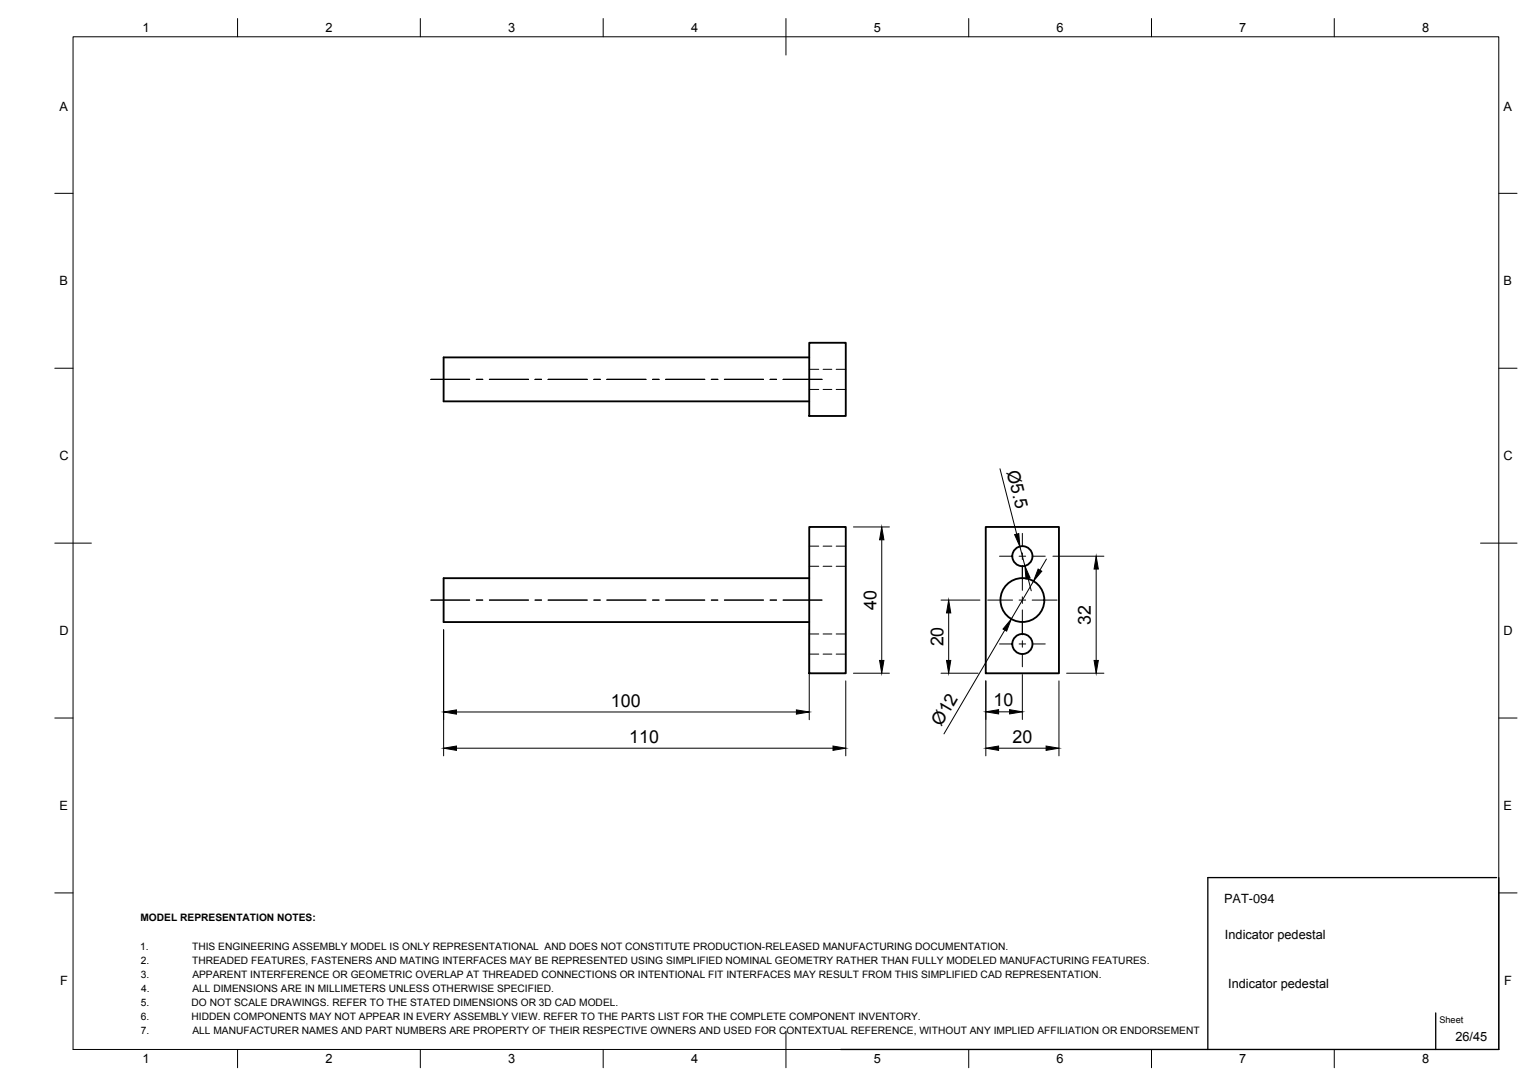
ISO-10303-21;
HEADER;
/* Generated by software containing ST-Developer
 * from STEP Tools, Inc. (www.steptools.com) 
 */

FILE_DESCRIPTION(
/* description */ ('Shaft runout checking stand'),
/* implementation_level */ '2;1');

FILE_NAME(
/* name */ 'Indicator pedestal.step',
/* time_stamp */ '2026-11-02T21:12:33-08:00',
/* author */ (''),
/* organization */ (''),
/* preprocessor_version */ 'ST-DEVELOPER v20.2',
/* originating_system */ 'Autodesk Translation Framework v15.17.0.0',
/* authorisation */ '');

FILE_SCHEMA (('AUTOMOTIVE_DESIGN { 1 0 10303 214 3 1 1 }'));
ENDSEC;

DATA;
#10=MECHANICAL_DESIGN_GEOMETRIC_PRESENTATION_REPRESENTATION('',(#486),#11748);
#400=SHAPE_REPRESENTATION_RELATIONSHIP('SRR','None',#11949,#443);
#443=ADVANCED_BREP_SHAPE_REPRESENTATION('',(#535),#11725);
#486=STYLED_ITEM('',(#12169),#535);
#535=MANIFOLD_SOLID_BREP('Body1',#6231);
#635=FACE_BOUND('',#1708,.T.);
#636=FACE_BOUND('',#1709,.T.);
#637=FACE_BOUND('',#1710,.T.);
#638=FACE_BOUND('',#1712,.T.);
#639=FACE_BOUND('',#1713,.T.);
#802=CIRCLE('',#7112,0.6);
#803=CIRCLE('',#7113,0.6);
#804=CIRCLE('',#7116,0.275);
#805=CIRCLE('',#7117,0.275);
#806=CIRCLE('',#7119,0.275);
#807=CIRCLE('',#7120,0.275);
#998=CYLINDRICAL_SURFACE('',#7111,0.6);
#999=CYLINDRICAL_SURFACE('',#7115,0.275);
#1000=CYLINDRICAL_SURFACE('',#7118,0.275);
#1258=FACE_OUTER_BOUND('',#1699,.T.);
#1259=FACE_OUTER_BOUND('',#1700,.T.);
#1260=FACE_OUTER_BOUND('',#1701,.T.);
#1261=FACE_OUTER_BOUND('',#1702,.T.);
#1262=FACE_OUTER_BOUND('',#1703,.T.);
#1263=FACE_OUTER_BOUND('',#1704,.T.);
#1264=FACE_OUTER_BOUND('',#1705,.T.);
#1265=FACE_OUTER_BOUND('',#1706,.T.);
#1266=FACE_OUTER_BOUND('',#1707,.T.);
#1267=FACE_OUTER_BOUND('',#1711,.T.);
#1699=EDGE_LOOP('',(#5040,#5041,#5042,#5043));
#1700=EDGE_LOOP('',(#5044));
#1701=EDGE_LOOP('',(#5045,#5046,#5047,#5048));
#1702=EDGE_LOOP('',(#5049,#5050,#5051,#5052));
#1703=EDGE_LOOP('',(#5053,#5054,#5055,#5056));
#1704=EDGE_LOOP('',(#5057,#5058,#5059,#5060));
#1705=EDGE_LOOP('',(#5061,#5062,#5063,#5064));
#1706=EDGE_LOOP('',(#5065,#5066,#5067,#5068));
#1707=EDGE_LOOP('',(#5069,#5070,#5071,#5072));
#1708=EDGE_LOOP('',(#5073));
#1709=EDGE_LOOP('',(#5074));
#1710=EDGE_LOOP('',(#5075));
#1711=EDGE_LOOP('',(#5076,#5077,#5078,#5079));
#1712=EDGE_LOOP('',(#5080));
#1713=EDGE_LOOP('',(#5081));
#2230=LINE('',#10516,#2697);
#2231=LINE('',#10523,#2698);
#2232=LINE('',#10529,#2699);
#2233=LINE('',#10534,#2700);
#2234=LINE('',#10536,#2701);
#2235=LINE('',#10538,#2702);
#2236=LINE('',#10539,#2703);
#2237=LINE('',#10542,#2704);
#2238=LINE('',#10544,#2705);
#2239=LINE('',#10545,#2706);
#2240=LINE('',#10548,#2707);
#2241=LINE('',#10550,#2708);
#2242=LINE('',#10551,#2709);
#2243=LINE('',#10553,#2710);
#2244=LINE('',#10554,#2711);
#2697=VECTOR('',#8595,0.6);
#2698=VECTOR('',#8604,0.275);
#2699=VECTOR('',#8611,0.275);
#2700=VECTOR('',#8616,1.);
#2701=VECTOR('',#8617,1.);
#2702=VECTOR('',#8618,1.);
#2703=VECTOR('',#8619,1.);
#2704=VECTOR('',#8622,1.);
#2705=VECTOR('',#8623,1.);
#2706=VECTOR('',#8624,1.);
#2707=VECTOR('',#8627,1.);
#2708=VECTOR('',#8628,1.);
#2709=VECTOR('',#8629,1.);
#2710=VECTOR('',#8632,1.);
#2711=VECTOR('',#8633,1.);
#3134=VERTEX_POINT('',#10513);
#3135=VERTEX_POINT('',#10515);
#3136=VERTEX_POINT('',#10520);
#3137=VERTEX_POINT('',#10522);
#3138=VERTEX_POINT('',#10526);
#3139=VERTEX_POINT('',#10528);
#3140=VERTEX_POINT('',#10532);
#3141=VERTEX_POINT('',#10533);
#3142=VERTEX_POINT('',#10535);
#3143=VERTEX_POINT('',#10537);
#3144=VERTEX_POINT('',#10541);
#3145=VERTEX_POINT('',#10543);
#3146=VERTEX_POINT('',#10547);
#3147=VERTEX_POINT('',#10549);
#3806=EDGE_CURVE('',#3134,#3134,#802,.T.);
#3807=EDGE_CURVE('',#3134,#3135,#2230,.T.);
#3808=EDGE_CURVE('',#3135,#3135,#803,.T.);
#3809=EDGE_CURVE('',#3136,#3136,#804,.T.);
#3810=EDGE_CURVE('',#3136,#3137,#2231,.T.);
#3811=EDGE_CURVE('',#3137,#3137,#805,.T.);
#3812=EDGE_CURVE('',#3138,#3138,#806,.T.);
#3813=EDGE_CURVE('',#3138,#3139,#2232,.T.);
#3814=EDGE_CURVE('',#3139,#3139,#807,.T.);
#3815=EDGE_CURVE('',#3140,#3141,#2233,.T.);
#3816=EDGE_CURVE('',#3141,#3142,#2234,.T.);
#3817=EDGE_CURVE('',#3143,#3142,#2235,.T.);
#3818=EDGE_CURVE('',#3140,#3143,#2236,.T.);
#3819=EDGE_CURVE('',#3144,#3140,#2237,.T.);
#3820=EDGE_CURVE('',#3145,#3143,#2238,.T.);
#3821=EDGE_CURVE('',#3144,#3145,#2239,.T.);
#3822=EDGE_CURVE('',#3146,#3144,#2240,.T.);
#3823=EDGE_CURVE('',#3147,#3145,#2241,.T.);
#3824=EDGE_CURVE('',#3146,#3147,#2242,.T.);
#3825=EDGE_CURVE('',#3141,#3146,#2243,.T.);
#3826=EDGE_CURVE('',#3142,#3147,#2244,.T.);
#5040=ORIENTED_EDGE('',*,*,#3806,.F.);
#5041=ORIENTED_EDGE('',*,*,#3807,.T.);
#5042=ORIENTED_EDGE('',*,*,#3808,.F.);
#5043=ORIENTED_EDGE('',*,*,#3807,.F.);
#5044=ORIENTED_EDGE('',*,*,#3806,.T.);
#5045=ORIENTED_EDGE('',*,*,#3809,.F.);
#5046=ORIENTED_EDGE('',*,*,#3810,.T.);
#5047=ORIENTED_EDGE('',*,*,#3811,.F.);
#5048=ORIENTED_EDGE('',*,*,#3810,.F.);
#5049=ORIENTED_EDGE('',*,*,#3812,.F.);
#5050=ORIENTED_EDGE('',*,*,#3813,.T.);
#5051=ORIENTED_EDGE('',*,*,#3814,.F.);
#5052=ORIENTED_EDGE('',*,*,#3813,.F.);
#5053=ORIENTED_EDGE('',*,*,#3815,.T.);
#5054=ORIENTED_EDGE('',*,*,#3816,.T.);
#5055=ORIENTED_EDGE('',*,*,#3817,.F.);
#5056=ORIENTED_EDGE('',*,*,#3818,.F.);
#5057=ORIENTED_EDGE('',*,*,#3819,.T.);
#5058=ORIENTED_EDGE('',*,*,#3818,.T.);
#5059=ORIENTED_EDGE('',*,*,#3820,.F.);
#5060=ORIENTED_EDGE('',*,*,#3821,.F.);
#5061=ORIENTED_EDGE('',*,*,#3822,.T.);
#5062=ORIENTED_EDGE('',*,*,#3821,.T.);
#5063=ORIENTED_EDGE('',*,*,#3823,.F.);
#5064=ORIENTED_EDGE('',*,*,#3824,.F.);
#5065=ORIENTED_EDGE('',*,*,#3825,.T.);
#5066=ORIENTED_EDGE('',*,*,#3824,.T.);
#5067=ORIENTED_EDGE('',*,*,#3826,.F.);
#5068=ORIENTED_EDGE('',*,*,#3816,.F.);
#5069=ORIENTED_EDGE('',*,*,#3826,.T.);
#5070=ORIENTED_EDGE('',*,*,#3823,.T.);
#5071=ORIENTED_EDGE('',*,*,#3820,.T.);
#5072=ORIENTED_EDGE('',*,*,#3817,.T.);
#5073=ORIENTED_EDGE('',*,*,#3808,.T.);
#5074=ORIENTED_EDGE('',*,*,#3811,.T.);
#5075=ORIENTED_EDGE('',*,*,#3814,.T.);
#5076=ORIENTED_EDGE('',*,*,#3825,.F.);
#5077=ORIENTED_EDGE('',*,*,#3815,.F.);
#5078=ORIENTED_EDGE('',*,*,#3819,.F.);
#5079=ORIENTED_EDGE('',*,*,#3822,.F.);
#5080=ORIENTED_EDGE('',*,*,#3809,.T.);
#5081=ORIENTED_EDGE('',*,*,#3812,.T.);
#5757=PLANE('',#7114);
#5758=PLANE('',#7121);
#5759=PLANE('',#7122);
#5760=PLANE('',#7123);
#5761=PLANE('',#7124);
#5762=PLANE('',#7125);
#5763=PLANE('',#7126);
#6058=ADVANCED_FACE('',(#1258),#998,.T.);
#6059=ADVANCED_FACE('',(#1259),#5757,.T.);
#6060=ADVANCED_FACE('',(#1260),#999,.F.);
#6061=ADVANCED_FACE('',(#1261),#1000,.F.);
#6062=ADVANCED_FACE('',(#1262),#5758,.T.);
#6063=ADVANCED_FACE('',(#1263),#5759,.T.);
#6064=ADVANCED_FACE('',(#1264),#5760,.T.);
#6065=ADVANCED_FACE('',(#1265),#5761,.T.);
#6066=ADVANCED_FACE('',(#1266,#635,#636,#637),#5762,.T.);
#6067=ADVANCED_FACE('',(#1267,#638,#639),#5763,.F.);
#6231=CLOSED_SHELL('',(#6058,#6059,#6060,#6061,#6062,#6063,#6064,#6065,
#6066,#6067));
#7110=AXIS2_PLACEMENT_3D('',#10511,#8589,#8590);
#7111=AXIS2_PLACEMENT_3D('',#10512,#8591,#8592);
#7112=AXIS2_PLACEMENT_3D('',#10514,#8593,#8594);
#7113=AXIS2_PLACEMENT_3D('',#10517,#8596,#8597);
#7114=AXIS2_PLACEMENT_3D('',#10518,#8598,#8599);
#7115=AXIS2_PLACEMENT_3D('',#10519,#8600,#8601);
#7116=AXIS2_PLACEMENT_3D('',#10521,#8602,#8603);
#7117=AXIS2_PLACEMENT_3D('',#10524,#8605,#8606);
#7118=AXIS2_PLACEMENT_3D('',#10525,#8607,#8608);
#7119=AXIS2_PLACEMENT_3D('',#10527,#8609,#8610);
#7120=AXIS2_PLACEMENT_3D('',#10530,#8612,#8613);
#7121=AXIS2_PLACEMENT_3D('',#10531,#8614,#8615);
#7122=AXIS2_PLACEMENT_3D('',#10540,#8620,#8621);
#7123=AXIS2_PLACEMENT_3D('',#10546,#8625,#8626);
#7124=AXIS2_PLACEMENT_3D('',#10552,#8630,#8631);
#7125=AXIS2_PLACEMENT_3D('',#10555,#8634,#8635);
#7126=AXIS2_PLACEMENT_3D('',#10556,#8636,#8637);
#8589=DIRECTION('axis',(0.,0.,1.));
#8590=DIRECTION('refdir',(1.,0.,0.));
#8591=DIRECTION('center_axis',(0.,0.,1.));
#8592=DIRECTION('ref_axis',(1.,0.,0.));
#8593=DIRECTION('center_axis',(0.,0.,1.));
#8594=DIRECTION('ref_axis',(1.,0.,0.));
#8595=DIRECTION('',(0.,0.,-1.));
#8596=DIRECTION('center_axis',(0.,0.,-1.));
#8597=DIRECTION('ref_axis',(1.,0.,0.));
#8598=DIRECTION('center_axis',(0.,0.,1.));
#8599=DIRECTION('ref_axis',(1.,0.,0.));
#8600=DIRECTION('center_axis',(0.,0.,1.));
#8601=DIRECTION('ref_axis',(1.,0.,0.));
#8602=DIRECTION('center_axis',(0.,0.,1.));
#8603=DIRECTION('ref_axis',(1.,0.,0.));
#8604=DIRECTION('',(0.,0.,1.));
#8605=DIRECTION('center_axis',(0.,0.,-1.));
#8606=DIRECTION('ref_axis',(1.,0.,0.));
#8607=DIRECTION('center_axis',(0.,0.,1.));
#8608=DIRECTION('ref_axis',(1.,0.,0.));
#8609=DIRECTION('center_axis',(0.,0.,1.));
#8610=DIRECTION('ref_axis',(1.,0.,0.));
#8611=DIRECTION('',(0.,0.,1.));
#8612=DIRECTION('center_axis',(0.,0.,-1.));
#8613=DIRECTION('ref_axis',(1.,0.,0.));
#8614=DIRECTION('center_axis',(0.,1.,0.));
#8615=DIRECTION('ref_axis',(-1.,0.,0.));
#8616=DIRECTION('',(-1.,0.,0.));
#8617=DIRECTION('',(0.,0.,1.));
#8618=DIRECTION('',(-1.,0.,0.));
#8619=DIRECTION('',(0.,0.,1.));
#8620=DIRECTION('center_axis',(1.,0.,0.));
#8621=DIRECTION('ref_axis',(0.,1.,0.));
#8622=DIRECTION('',(0.,1.,0.));
#8623=DIRECTION('',(0.,1.,0.));
#8624=DIRECTION('',(0.,0.,1.));
#8625=DIRECTION('center_axis',(0.,-1.,0.));
#8626=DIRECTION('ref_axis',(1.,0.,0.));
#8627=DIRECTION('',(1.,0.,0.));
#8628=DIRECTION('',(1.,0.,0.));
#8629=DIRECTION('',(0.,0.,1.));
#8630=DIRECTION('center_axis',(-1.,0.,0.));
#8631=DIRECTION('ref_axis',(0.,-1.,0.));
#8632=DIRECTION('',(0.,-1.,0.));
#8633=DIRECTION('',(0.,-1.,0.));
#8634=DIRECTION('center_axis',(0.,0.,1.));
#8635=DIRECTION('ref_axis',(1.,0.,0.));
#8636=DIRECTION('center_axis',(0.,0.,1.));
#8637=DIRECTION('ref_axis',(1.,0.,0.));
#10511=CARTESIAN_POINT('',(0.,0.,0.));
#10512=CARTESIAN_POINT('Origin',(5.,0.,3.8));
#10513=CARTESIAN_POINT('',(4.4,-7.34788079488412E-17,13.8));
#10514=CARTESIAN_POINT('Origin',(5.,0.,13.8));
#10515=CARTESIAN_POINT('',(4.4,-7.34788079488412E-17,3.8));
#10516=CARTESIAN_POINT('',(4.4,-7.34788079488412E-17,3.8));
#10517=CARTESIAN_POINT('Origin',(5.,0.,3.8));
#10518=CARTESIAN_POINT('Origin',(5.,0.,13.8));
#10519=CARTESIAN_POINT('Origin',(5.,-1.2,2.7));
#10520=CARTESIAN_POINT('',(4.725,-1.2,2.8));
#10521=CARTESIAN_POINT('Origin',(5.,-1.2,2.8));
#10522=CARTESIAN_POINT('',(4.725,-1.2,3.8));
#10523=CARTESIAN_POINT('',(4.725,-1.2,2.7));
#10524=CARTESIAN_POINT('Origin',(5.,-1.2,3.8));
#10525=CARTESIAN_POINT('Origin',(5.,1.2,2.7));
#10526=CARTESIAN_POINT('',(4.725,1.2,2.8));
#10527=CARTESIAN_POINT('Origin',(5.,1.2,2.8));
#10528=CARTESIAN_POINT('',(4.725,1.2,3.8));
#10529=CARTESIAN_POINT('',(4.725,1.2,2.7));
#10530=CARTESIAN_POINT('Origin',(5.,1.2,3.8));
#10531=CARTESIAN_POINT('Origin',(6.,2.,2.8));
#10532=CARTESIAN_POINT('',(6.,2.,2.8));
#10533=CARTESIAN_POINT('',(4.,2.,2.8));
#10534=CARTESIAN_POINT('',(6.,2.,2.8));
#10535=CARTESIAN_POINT('',(4.,2.,3.8));
#10536=CARTESIAN_POINT('',(4.,2.,2.8));
#10537=CARTESIAN_POINT('',(6.,2.,3.8));
#10538=CARTESIAN_POINT('',(6.,2.,3.8));
#10539=CARTESIAN_POINT('',(6.,2.,2.8));
#10540=CARTESIAN_POINT('Origin',(6.,-2.,2.8));
#10541=CARTESIAN_POINT('',(6.,-2.,2.8));
#10542=CARTESIAN_POINT('',(6.,-2.,2.8));
#10543=CARTESIAN_POINT('',(6.,-2.,3.8));
#10544=CARTESIAN_POINT('',(6.,-2.,3.8));
#10545=CARTESIAN_POINT('',(6.,-2.,2.8));
#10546=CARTESIAN_POINT('Origin',(4.,-2.,2.8));
#10547=CARTESIAN_POINT('',(4.,-2.,2.8));
#10548=CARTESIAN_POINT('',(4.,-2.,2.8));
#10549=CARTESIAN_POINT('',(4.,-2.,3.8));
#10550=CARTESIAN_POINT('',(4.,-2.,3.8));
#10551=CARTESIAN_POINT('',(4.,-2.,2.8));
#10552=CARTESIAN_POINT('Origin',(4.,2.,2.8));
#10553=CARTESIAN_POINT('',(4.,2.,2.8));
#10554=CARTESIAN_POINT('',(4.,2.,3.8));
#10555=CARTESIAN_POINT('Origin',(5.,0.,3.8));
#10556=CARTESIAN_POINT('Origin',(5.,0.,2.8));
#11676=UNCERTAINTY_MEASURE_WITH_UNIT(LENGTH_MEASURE(0.001),#11749,
'DISTANCE_ACCURACY_VALUE',
'Maximum model space distance between geometric entities at asserted c
onnectivities');
#11699=UNCERTAINTY_MEASURE_WITH_UNIT(LENGTH_MEASURE(0.001),#11749,
'DISTANCE_ACCURACY_VALUE',
'Maximum model space distance between geometric entities at asserted c
onnectivities');
#11725=(
GEOMETRIC_REPRESENTATION_CONTEXT(3)
GLOBAL_UNCERTAINTY_ASSIGNED_CONTEXT((#11676))
GLOBAL_UNIT_ASSIGNED_CONTEXT((#11749,#11751,#11752))
REPRESENTATION_CONTEXT('','3D')
);
#11748=(
GEOMETRIC_REPRESENTATION_CONTEXT(3)
GLOBAL_UNCERTAINTY_ASSIGNED_CONTEXT((#11699))
GLOBAL_UNIT_ASSIGNED_CONTEXT((#11749,#11751,#11752))
REPRESENTATION_CONTEXT('','3D')
);
#11749=(
LENGTH_UNIT()
NAMED_UNIT(*)
SI_UNIT(.CENTI.,.METRE.)
);
#11751=(
NAMED_UNIT(*)
PLANE_ANGLE_UNIT()
SI_UNIT($,.RADIAN.)
);
#11752=(
NAMED_UNIT(*)
SI_UNIT($,.STERADIAN.)
SOLID_ANGLE_UNIT()
);
#11778=SHAPE_DEFINITION_REPRESENTATION(#11826,#11949);
#11826=PRODUCT_DEFINITION_SHAPE('',$,#11998);
#11949=SHAPE_REPRESENTATION('',(#7110),#11725);
#11972=PRODUCT_DEFINITION_CONTEXT('part definition',#12118,'design');
#11998=PRODUCT_DEFINITION('Indicator pedestal','Indicator pedestal',#12046,
#11972);
#12046=PRODUCT_DEFINITION_FORMATION('',$,#12145);
#12118=APPLICATION_CONTEXT(
'Core Data for Automotive Mechanical Design Process');
#12119=PRODUCT_CONTEXT('part definition',#12118,'mechanical');
#12145=PRODUCT('Indicator pedestal','Indicator pedestal',
'Indicator pedestal',(#12119));
#12169=PRESENTATION_STYLE_ASSIGNMENT((#12174));
#12174=SURFACE_STYLE_USAGE(.BOTH.,#12179);
#12179=SURFACE_SIDE_STYLE('',(#12184));
#12184=SURFACE_STYLE_FILL_AREA(#12189);
#12189=FILL_AREA_STYLE('CAD Library Painted - Engineering blue',(#12194));
#12194=FILL_AREA_STYLE_COLOUR('CAD Library Painted - Engineering blue',
#12199);
#12199=COLOUR_RGB('CAD Library Painted - Engineering blue',0.12156862745098,
0.356862745098039,0.6);
ENDSEC;
END-ISO-10303-21;
